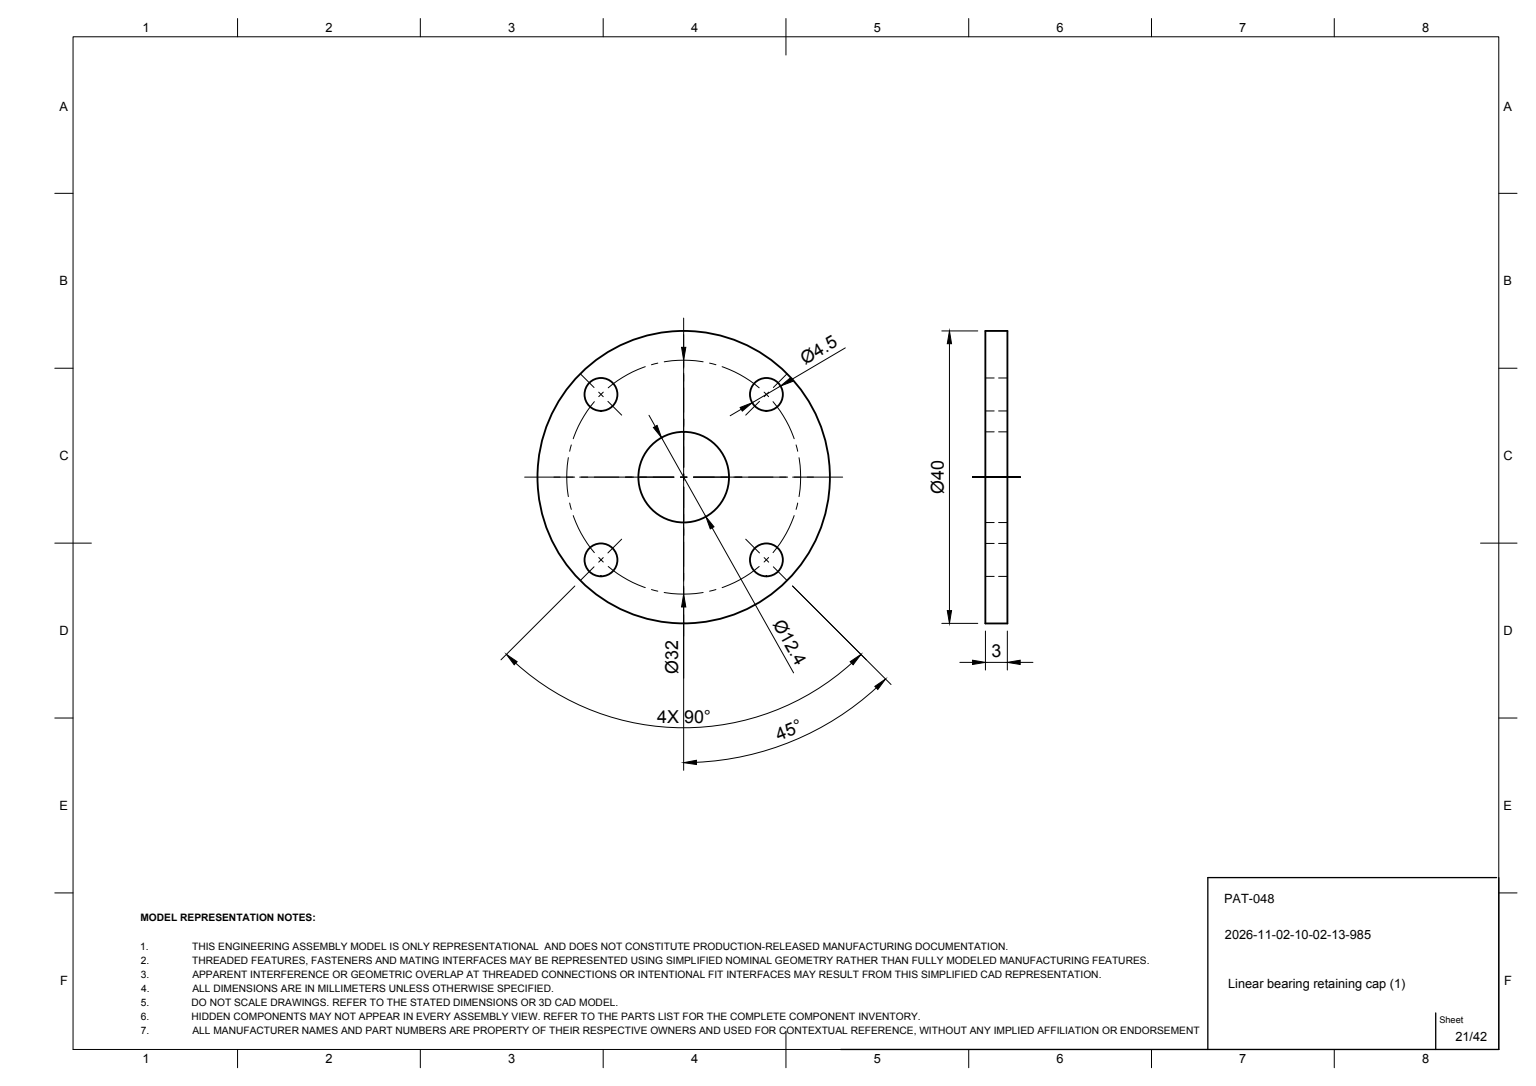
ISO-10303-21;
HEADER;
/* Generated by software containing ST-Developer
 * from STEP Tools, Inc. (www.steptools.com) 
 */

FILE_DESCRIPTION(
/* description */ ('Guided pneumatic stop gate'),
/* implementation_level */ '2;1');

FILE_NAME(
/* name */ 'Linear bearing retaining cap (1).step',
/* time_stamp */ '2026-10-27T21:43:45-07:00',
/* author */ (''),
/* organization */ (''),
/* preprocessor_version */ 'ST-DEVELOPER v20.2',
/* originating_system */ 'Autodesk Translation Framework v15.17.0.0',
/* authorisation */ '');

FILE_SCHEMA (('AUTOMOTIVE_DESIGN { 1 0 10303 214 3 1 1 }'));
ENDSEC;

DATA;
#10=MECHANICAL_DESIGN_GEOMETRIC_PRESENTATION_REPRESENTATION('',(#556),#14392);
#472=SHAPE_REPRESENTATION_RELATIONSHIP('SRR','None',#14607,#514);
#514=ADVANCED_BREP_SHAPE_REPRESENTATION('',(#597),#14369);
#556=STYLED_ITEM('',(#14891),#597);
#597=MANIFOLD_SOLID_BREP('Body1',#7897);
#747=FACE_BOUND('',#2006,.T.);
#748=FACE_BOUND('',#2007,.T.);
#749=FACE_BOUND('',#2008,.T.);
#750=FACE_BOUND('',#2009,.T.);
#751=FACE_BOUND('',#2010,.T.);
#752=FACE_BOUND('',#2012,.T.);
#753=FACE_BOUND('',#2013,.T.);
#754=FACE_BOUND('',#2014,.T.);
#755=FACE_BOUND('',#2015,.T.);
#756=FACE_BOUND('',#2016,.T.);
#997=PLANE('',#8936);
#998=PLANE('',#8937);
#1392=FACE_OUTER_BOUND('',#1999,.T.);
#1393=FACE_OUTER_BOUND('',#2000,.T.);
#1394=FACE_OUTER_BOUND('',#2001,.T.);
#1395=FACE_OUTER_BOUND('',#2002,.T.);
#1396=FACE_OUTER_BOUND('',#2003,.T.);
#1397=FACE_OUTER_BOUND('',#2004,.T.);
#1398=FACE_OUTER_BOUND('',#2005,.T.);
#1399=FACE_OUTER_BOUND('',#2011,.T.);
#1999=EDGE_LOOP('',(#6438,#6439,#6440,#6441));
#2000=EDGE_LOOP('',(#6442,#6443,#6444,#6445));
#2001=EDGE_LOOP('',(#6446,#6447,#6448,#6449));
#2002=EDGE_LOOP('',(#6450,#6451,#6452,#6453));
#2003=EDGE_LOOP('',(#6454,#6455,#6456,#6457));
#2004=EDGE_LOOP('',(#6458,#6459,#6460,#6461));
#2005=EDGE_LOOP('',(#6462));
#2006=EDGE_LOOP('',(#6463));
#2007=EDGE_LOOP('',(#6464));
#2008=EDGE_LOOP('',(#6465));
#2009=EDGE_LOOP('',(#6466));
#2010=EDGE_LOOP('',(#6467));
#2011=EDGE_LOOP('',(#6468));
#2012=EDGE_LOOP('',(#6469));
#2013=EDGE_LOOP('',(#6470));
#2014=EDGE_LOOP('',(#6471));
#2015=EDGE_LOOP('',(#6472));
#2016=EDGE_LOOP('',(#6473));
#2594=LINE('',#13169,#3139);
#2595=LINE('',#13175,#3140);
#2596=LINE('',#13181,#3141);
#2597=LINE('',#13187,#3142);
#2598=LINE('',#13193,#3143);
#2599=LINE('',#13199,#3144);
#3139=VECTOR('',#10769,0.225);
#3140=VECTOR('',#10776,0.225);
#3141=VECTOR('',#10783,0.225);
#3142=VECTOR('',#10790,0.225);
#3143=VECTOR('',#10797,0.62);
#3144=VECTOR('',#10804,2.);
#3587=CIRCLE('',#8919,0.225);
#3588=CIRCLE('',#8920,0.225);
#3589=CIRCLE('',#8922,0.225);
#3590=CIRCLE('',#8923,0.225);
#3591=CIRCLE('',#8925,0.225);
#3592=CIRCLE('',#8926,0.225);
#3593=CIRCLE('',#8928,0.225);
#3594=CIRCLE('',#8929,0.225);
#3595=CIRCLE('',#8931,0.62);
#3596=CIRCLE('',#8932,0.62);
#3597=CIRCLE('',#8934,2.);
#3598=CIRCLE('',#8935,2.);
#4096=VERTEX_POINT('',#13166);
#4097=VERTEX_POINT('',#13168);
#4098=VERTEX_POINT('',#13172);
#4099=VERTEX_POINT('',#13174);
#4100=VERTEX_POINT('',#13178);
#4101=VERTEX_POINT('',#13180);
#4102=VERTEX_POINT('',#13184);
#4103=VERTEX_POINT('',#13186);
#4104=VERTEX_POINT('',#13190);
#4105=VERTEX_POINT('',#13192);
#4106=VERTEX_POINT('',#13196);
#4107=VERTEX_POINT('',#13198);
#4917=EDGE_CURVE('',#4096,#4096,#3587,.T.);
#4918=EDGE_CURVE('',#4096,#4097,#2594,.T.);
#4919=EDGE_CURVE('',#4097,#4097,#3588,.T.);
#4920=EDGE_CURVE('',#4098,#4098,#3589,.T.);
#4921=EDGE_CURVE('',#4098,#4099,#2595,.T.);
#4922=EDGE_CURVE('',#4099,#4099,#3590,.T.);
#4923=EDGE_CURVE('',#4100,#4100,#3591,.T.);
#4924=EDGE_CURVE('',#4100,#4101,#2596,.T.);
#4925=EDGE_CURVE('',#4101,#4101,#3592,.T.);
#4926=EDGE_CURVE('',#4102,#4102,#3593,.T.);
#4927=EDGE_CURVE('',#4102,#4103,#2597,.T.);
#4928=EDGE_CURVE('',#4103,#4103,#3594,.T.);
#4929=EDGE_CURVE('',#4104,#4104,#3595,.T.);
#4930=EDGE_CURVE('',#4104,#4105,#2598,.T.);
#4931=EDGE_CURVE('',#4105,#4105,#3596,.T.);
#4932=EDGE_CURVE('',#4106,#4106,#3597,.T.);
#4933=EDGE_CURVE('',#4106,#4107,#2599,.T.);
#4934=EDGE_CURVE('',#4107,#4107,#3598,.T.);
#6438=ORIENTED_EDGE('',*,*,#4917,.F.);
#6439=ORIENTED_EDGE('',*,*,#4918,.T.);
#6440=ORIENTED_EDGE('',*,*,#4919,.F.);
#6441=ORIENTED_EDGE('',*,*,#4918,.F.);
#6442=ORIENTED_EDGE('',*,*,#4920,.F.);
#6443=ORIENTED_EDGE('',*,*,#4921,.T.);
#6444=ORIENTED_EDGE('',*,*,#4922,.F.);
#6445=ORIENTED_EDGE('',*,*,#4921,.F.);
#6446=ORIENTED_EDGE('',*,*,#4923,.F.);
#6447=ORIENTED_EDGE('',*,*,#4924,.T.);
#6448=ORIENTED_EDGE('',*,*,#4925,.F.);
#6449=ORIENTED_EDGE('',*,*,#4924,.F.);
#6450=ORIENTED_EDGE('',*,*,#4926,.F.);
#6451=ORIENTED_EDGE('',*,*,#4927,.T.);
#6452=ORIENTED_EDGE('',*,*,#4928,.F.);
#6453=ORIENTED_EDGE('',*,*,#4927,.F.);
#6454=ORIENTED_EDGE('',*,*,#4929,.F.);
#6455=ORIENTED_EDGE('',*,*,#4930,.T.);
#6456=ORIENTED_EDGE('',*,*,#4931,.T.);
#6457=ORIENTED_EDGE('',*,*,#4930,.F.);
#6458=ORIENTED_EDGE('',*,*,#4932,.F.);
#6459=ORIENTED_EDGE('',*,*,#4933,.T.);
#6460=ORIENTED_EDGE('',*,*,#4934,.T.);
#6461=ORIENTED_EDGE('',*,*,#4933,.F.);
#6462=ORIENTED_EDGE('',*,*,#4932,.T.);
#6463=ORIENTED_EDGE('',*,*,#4929,.T.);
#6464=ORIENTED_EDGE('',*,*,#4928,.T.);
#6465=ORIENTED_EDGE('',*,*,#4925,.T.);
#6466=ORIENTED_EDGE('',*,*,#4922,.T.);
#6467=ORIENTED_EDGE('',*,*,#4919,.T.);
#6468=ORIENTED_EDGE('',*,*,#4934,.F.);
#6469=ORIENTED_EDGE('',*,*,#4931,.F.);
#6470=ORIENTED_EDGE('',*,*,#4926,.T.);
#6471=ORIENTED_EDGE('',*,*,#4923,.T.);
#6472=ORIENTED_EDGE('',*,*,#4920,.T.);
#6473=ORIENTED_EDGE('',*,*,#4917,.T.);
#7339=CYLINDRICAL_SURFACE('',#8918,0.225);
#7340=CYLINDRICAL_SURFACE('',#8921,0.225);
#7341=CYLINDRICAL_SURFACE('',#8924,0.225);
#7342=CYLINDRICAL_SURFACE('',#8927,0.225);
#7343=CYLINDRICAL_SURFACE('',#8930,0.62);
#7344=CYLINDRICAL_SURFACE('',#8933,2.);
#7674=ADVANCED_FACE('',(#1392),#7339,.F.);
#7675=ADVANCED_FACE('',(#1393),#7340,.F.);
#7676=ADVANCED_FACE('',(#1394),#7341,.F.);
#7677=ADVANCED_FACE('',(#1395),#7342,.F.);
#7678=ADVANCED_FACE('',(#1396),#7343,.F.);
#7679=ADVANCED_FACE('',(#1397),#7344,.T.);
#7680=ADVANCED_FACE('',(#1398,#747,#748,#749,#750,#751),#997,.T.);
#7681=ADVANCED_FACE('',(#1399,#752,#753,#754,#755,#756),#998,.F.);
#7897=CLOSED_SHELL('',(#7674,#7675,#7676,#7677,#7678,#7679,#7680,#7681));
#8917=AXIS2_PLACEMENT_3D('',#13164,#10763,#10764);
#8918=AXIS2_PLACEMENT_3D('',#13165,#10765,#10766);
#8919=AXIS2_PLACEMENT_3D('',#13167,#10767,#10768);
#8920=AXIS2_PLACEMENT_3D('',#13170,#10770,#10771);
#8921=AXIS2_PLACEMENT_3D('',#13171,#10772,#10773);
#8922=AXIS2_PLACEMENT_3D('',#13173,#10774,#10775);
#8923=AXIS2_PLACEMENT_3D('',#13176,#10777,#10778);
#8924=AXIS2_PLACEMENT_3D('',#13177,#10779,#10780);
#8925=AXIS2_PLACEMENT_3D('',#13179,#10781,#10782);
#8926=AXIS2_PLACEMENT_3D('',#13182,#10784,#10785);
#8927=AXIS2_PLACEMENT_3D('',#13183,#10786,#10787);
#8928=AXIS2_PLACEMENT_3D('',#13185,#10788,#10789);
#8929=AXIS2_PLACEMENT_3D('',#13188,#10791,#10792);
#8930=AXIS2_PLACEMENT_3D('',#13189,#10793,#10794);
#8931=AXIS2_PLACEMENT_3D('',#13191,#10795,#10796);
#8932=AXIS2_PLACEMENT_3D('',#13194,#10798,#10799);
#8933=AXIS2_PLACEMENT_3D('',#13195,#10800,#10801);
#8934=AXIS2_PLACEMENT_3D('',#13197,#10802,#10803);
#8935=AXIS2_PLACEMENT_3D('',#13200,#10805,#10806);
#8936=AXIS2_PLACEMENT_3D('',#13201,#10807,#10808);
#8937=AXIS2_PLACEMENT_3D('',#13202,#10809,#10810);
#10763=DIRECTION('axis',(0.,0.,1.));
#10764=DIRECTION('refdir',(1.,0.,0.));
#10765=DIRECTION('center_axis',(0.,1.,0.));
#10766=DIRECTION('ref_axis',(1.,0.,0.));
#10767=DIRECTION('center_axis',(0.,1.,0.));
#10768=DIRECTION('ref_axis',(1.,0.,0.));
#10769=DIRECTION('',(0.,1.,0.));
#10770=DIRECTION('center_axis',(0.,-1.,0.));
#10771=DIRECTION('ref_axis',(1.,0.,0.));
#10772=DIRECTION('center_axis',(0.,1.,0.));
#10773=DIRECTION('ref_axis',(1.,0.,0.));
#10774=DIRECTION('center_axis',(0.,1.,0.));
#10775=DIRECTION('ref_axis',(1.,0.,0.));
#10776=DIRECTION('',(0.,1.,0.));
#10777=DIRECTION('center_axis',(0.,-1.,0.));
#10778=DIRECTION('ref_axis',(1.,0.,0.));
#10779=DIRECTION('center_axis',(0.,1.,0.));
#10780=DIRECTION('ref_axis',(1.,0.,0.));
#10781=DIRECTION('center_axis',(0.,1.,0.));
#10782=DIRECTION('ref_axis',(1.,0.,0.));
#10783=DIRECTION('',(0.,1.,0.));
#10784=DIRECTION('center_axis',(0.,-1.,0.));
#10785=DIRECTION('ref_axis',(1.,0.,0.));
#10786=DIRECTION('center_axis',(0.,1.,0.));
#10787=DIRECTION('ref_axis',(1.,0.,0.));
#10788=DIRECTION('center_axis',(0.,1.,0.));
#10789=DIRECTION('ref_axis',(1.,0.,0.));
#10790=DIRECTION('',(0.,1.,0.));
#10791=DIRECTION('center_axis',(0.,-1.,0.));
#10792=DIRECTION('ref_axis',(1.,0.,0.));
#10793=DIRECTION('center_axis',(0.,1.,0.));
#10794=DIRECTION('ref_axis',(1.,0.,0.));
#10795=DIRECTION('center_axis',(0.,-1.,0.));
#10796=DIRECTION('ref_axis',(1.,0.,0.));
#10797=DIRECTION('',(0.,-1.,0.));
#10798=DIRECTION('center_axis',(0.,-1.,0.));
#10799=DIRECTION('ref_axis',(1.,0.,0.));
#10800=DIRECTION('center_axis',(0.,1.,0.));
#10801=DIRECTION('ref_axis',(1.,0.,0.));
#10802=DIRECTION('center_axis',(0.,1.,0.));
#10803=DIRECTION('ref_axis',(1.,0.,0.));
#10804=DIRECTION('',(0.,-1.,0.));
#10805=DIRECTION('center_axis',(0.,1.,0.));
#10806=DIRECTION('ref_axis',(1.,0.,0.));
#10807=DIRECTION('center_axis',(0.,1.,0.));
#10808=DIRECTION('ref_axis',(1.,0.,0.));
#10809=DIRECTION('center_axis',(0.,1.,0.));
#10810=DIRECTION('ref_axis',(1.,0.,0.));
#13164=CARTESIAN_POINT('',(0.,0.,0.));
#13165=CARTESIAN_POINT('Origin',(-6.13137084989848,8.9,3.36862915010152));
#13166=CARTESIAN_POINT('',(-6.35637084989848,9.,3.36862915010152));
#13167=CARTESIAN_POINT('Origin',(-6.13137084989848,9.,3.36862915010152));
#13168=CARTESIAN_POINT('',(-6.35637084989848,9.3,3.36862915010152));
#13169=CARTESIAN_POINT('',(-6.35637084989848,8.9,3.36862915010152));
#13170=CARTESIAN_POINT('Origin',(-6.13137084989848,9.3,3.36862915010152));
#13171=CARTESIAN_POINT('Origin',(-6.13137084989848,8.9,5.63137084989848));
#13172=CARTESIAN_POINT('',(-6.35637084989848,9.,5.63137084989848));
#13173=CARTESIAN_POINT('Origin',(-6.13137084989848,9.,5.63137084989848));
#13174=CARTESIAN_POINT('',(-6.35637084989848,9.3,5.63137084989848));
#13175=CARTESIAN_POINT('',(-6.35637084989848,8.9,5.63137084989848));
#13176=CARTESIAN_POINT('Origin',(-6.13137084989848,9.3,5.63137084989848));
#13177=CARTESIAN_POINT('Origin',(-3.86862915010152,8.9,5.63137084989848));
#13178=CARTESIAN_POINT('',(-4.09362915010152,9.,5.63137084989848));
#13179=CARTESIAN_POINT('Origin',(-3.86862915010152,9.,5.63137084989848));
#13180=CARTESIAN_POINT('',(-4.09362915010152,9.3,5.63137084989848));
#13181=CARTESIAN_POINT('',(-4.09362915010152,8.9,5.63137084989848));
#13182=CARTESIAN_POINT('Origin',(-3.86862915010152,9.3,5.63137084989848));
#13183=CARTESIAN_POINT('Origin',(-3.86862915010152,8.9,3.36862915010152));
#13184=CARTESIAN_POINT('',(-4.09362915010152,9.,3.36862915010152));
#13185=CARTESIAN_POINT('Origin',(-3.86862915010152,9.,3.36862915010152));
#13186=CARTESIAN_POINT('',(-4.09362915010152,9.3,3.36862915010152));
#13187=CARTESIAN_POINT('',(-4.09362915010152,8.9,3.36862915010152));
#13188=CARTESIAN_POINT('Origin',(-3.86862915010152,9.3,3.36862915010152));
#13189=CARTESIAN_POINT('Origin',(-5.,9.,4.5));
#13190=CARTESIAN_POINT('',(-5.62,9.3,4.5));
#13191=CARTESIAN_POINT('Origin',(-5.,9.3,4.5));
#13192=CARTESIAN_POINT('',(-5.62,9.,4.5));
#13193=CARTESIAN_POINT('',(-5.62,9.,4.5));
#13194=CARTESIAN_POINT('Origin',(-5.,9.,4.5));
#13195=CARTESIAN_POINT('Origin',(-5.,9.,4.5));
#13196=CARTESIAN_POINT('',(-7.,9.3,4.5));
#13197=CARTESIAN_POINT('Origin',(-5.,9.3,4.5));
#13198=CARTESIAN_POINT('',(-7.,9.,4.5));
#13199=CARTESIAN_POINT('',(-7.,9.,4.5));
#13200=CARTESIAN_POINT('Origin',(-5.,9.,4.5));
#13201=CARTESIAN_POINT('Origin',(-5.,9.3,4.5));
#13202=CARTESIAN_POINT('Origin',(-5.,9.,4.5));
#14321=UNCERTAINTY_MEASURE_WITH_UNIT(LENGTH_MEASURE(0.001),#14393,
'DISTANCE_ACCURACY_VALUE',
'Maximum model space distance between geometric entities at asserted c
onnectivities');
#14344=UNCERTAINTY_MEASURE_WITH_UNIT(LENGTH_MEASURE(0.001),#14393,
'DISTANCE_ACCURACY_VALUE',
'Maximum model space distance between geometric entities at asserted c
onnectivities');
#14369=(
GEOMETRIC_REPRESENTATION_CONTEXT(3)
GLOBAL_UNCERTAINTY_ASSIGNED_CONTEXT((#14321))
GLOBAL_UNIT_ASSIGNED_CONTEXT((#14393,#14395,#14396))
REPRESENTATION_CONTEXT('','3D')
);
#14392=(
GEOMETRIC_REPRESENTATION_CONTEXT(3)
GLOBAL_UNCERTAINTY_ASSIGNED_CONTEXT((#14344))
GLOBAL_UNIT_ASSIGNED_CONTEXT((#14393,#14395,#14396))
REPRESENTATION_CONTEXT('','3D')
);
#14393=(
LENGTH_UNIT()
NAMED_UNIT(*)
SI_UNIT(.CENTI.,.METRE.)
);
#14395=(
NAMED_UNIT(*)
PLANE_ANGLE_UNIT()
SI_UNIT($,.RADIAN.)
);
#14396=(
NAMED_UNIT(*)
SI_UNIT($,.STERADIAN.)
SOLID_ANGLE_UNIT()
);
#14421=SHAPE_DEFINITION_REPRESENTATION(#14470,#14607);
#14470=PRODUCT_DEFINITION_SHAPE('',$,#14655);
#14607=SHAPE_REPRESENTATION('',(#8917),#14369);
#14630=PRODUCT_DEFINITION_CONTEXT('part definition',#14773,'design');
#14655=PRODUCT_DEFINITION('Linear bearing retaining cap (1)',
'Linear bearing retaining cap (1)',#14702,#14630);
#14702=PRODUCT_DEFINITION_FORMATION('',$,#14799);
#14773=APPLICATION_CONTEXT(
'Core Data for Automotive Mechanical Design Process');
#14774=PRODUCT_CONTEXT('part definition',#14773,'mechanical');
#14799=PRODUCT('Linear bearing retaining cap (1)',
'Linear bearing retaining cap (1)','Linear bearing retaining cap (1)',(#14774));
#14885=COLOUR_RGB('Grey',0.48,0.52,0.57);
#14886=FILL_AREA_STYLE_COLOUR('',#14885);
#14887=FILL_AREA_STYLE('',(#14886));
#14888=SURFACE_STYLE_FILL_AREA(#14887);
#14889=SURFACE_SIDE_STYLE('',(#14888));
#14890=SURFACE_STYLE_USAGE(.BOTH.,#14889);
#14891=PRESENTATION_STYLE_ASSIGNMENT((#14890));
ENDSEC;
END-ISO-10303-21;
